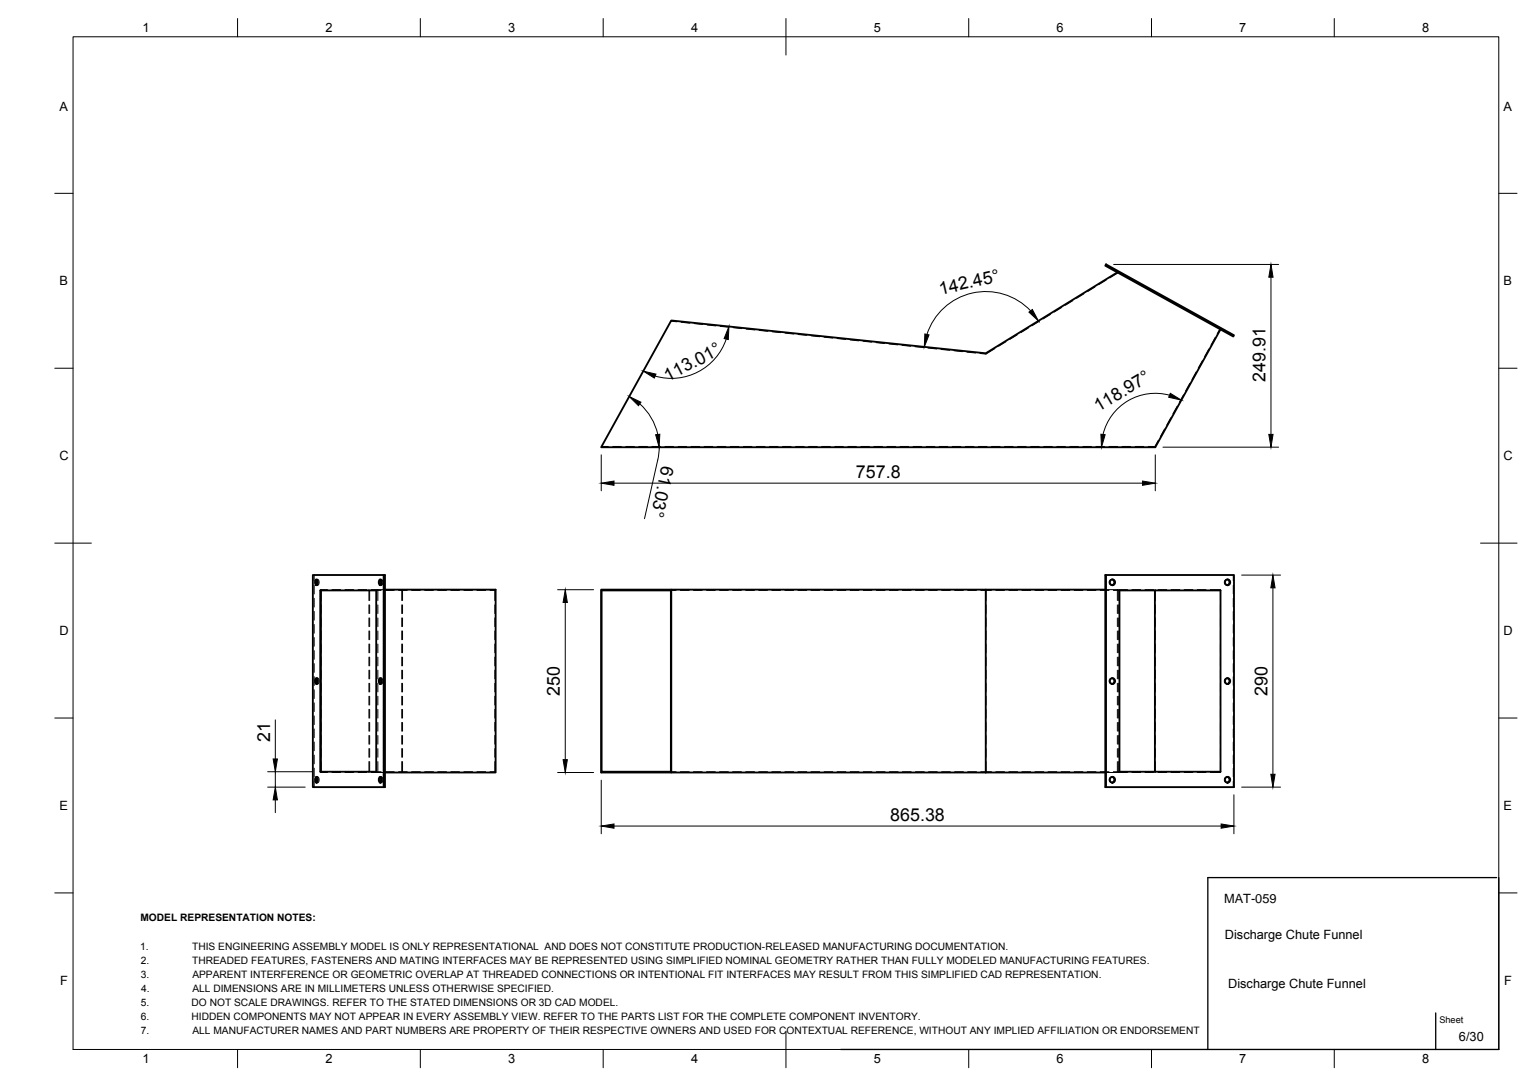
ISO-10303-21;
HEADER;
/* Generated by software containing ST-Developer
 * from STEP Tools, Inc. (www.steptools.com) 
 */

FILE_DESCRIPTION(
/* description */ ('', 'CAx-IF Rec.Pracs.---Representation and Presentation of Product Manufa
cturing Information (PMI)---4.0---2014-10-13'),
/* implementation_level */ '2;1');

FILE_NAME(
/* name */ 'Discharge Chute Funnel.step',
/* time_stamp */ '2026-10-28T23:00:48+01:00',
/* author */ (''),
/* organization */ (''),
/* preprocessor_version */ 'ST-DEVELOPER v20.2',
/* originating_system */ 'Autodesk Translation Framework v15.17.0.0',
/* authorisation */ '');

FILE_SCHEMA (('AP242_MANAGED_MODEL_BASED_3D_ENGINEERING_MIM_LF { 1 0 10303 442 2 1 4 }'));
ENDSEC;

DATA;
#10=MECHANICAL_DESIGN_GEOMETRIC_PRESENTATION_REPRESENTATION('',(#968),#61811);
#918=SHAPE_REPRESENTATION_RELATIONSHIP('SRR','None',#61976,#943);
#943=ADVANCED_BREP_SHAPE_REPRESENTATION('',(#1007),#61789);
#968=STYLED_ITEM('',(#62149),#1007);
#1007=MANIFOLD_SOLID_BREP('Body1',#33798);
#1101=CYLINDRICAL_SURFACE('',#34529,4.);
#1102=CYLINDRICAL_SURFACE('',#34532,4.);
#1103=CYLINDRICAL_SURFACE('',#34535,4.);
#1104=CYLINDRICAL_SURFACE('',#34538,4.);
#1105=CYLINDRICAL_SURFACE('',#34541,4.);
#1106=CYLINDRICAL_SURFACE('',#34544,4.);
#1908=FACE_BOUND('',#6367,.T.);
#1909=FACE_BOUND('',#6368,.T.);
#1910=FACE_BOUND('',#6369,.T.);
#1911=FACE_BOUND('',#6370,.T.);
#1912=FACE_BOUND('',#6371,.T.);
#1913=FACE_BOUND('',#6372,.T.);
#1914=FACE_BOUND('',#6373,.T.);
#1915=FACE_BOUND('',#6389,.T.);
#1916=FACE_BOUND('',#6390,.T.);
#1917=FACE_BOUND('',#6391,.T.);
#1918=FACE_BOUND('',#6392,.T.);
#1919=FACE_BOUND('',#6393,.T.);
#1920=FACE_BOUND('',#6394,.T.);
#1921=FACE_BOUND('',#6395,.T.);
#1922=FACE_BOUND('',#6399,.T.);
#2436=CIRCLE('',#34530,4.);
#2437=CIRCLE('',#34531,4.);
#2438=CIRCLE('',#34533,4.);
#2439=CIRCLE('',#34534,4.);
#2440=CIRCLE('',#34536,4.);
#2441=CIRCLE('',#34537,4.);
#2442=CIRCLE('',#34539,4.);
#2443=CIRCLE('',#34540,4.);
#2444=CIRCLE('',#34542,4.);
#2445=CIRCLE('',#34543,4.);
#2446=CIRCLE('',#34545,4.);
#2447=CIRCLE('',#34546,4.);
#4452=FACE_OUTER_BOUND('',#6360,.T.);
#4453=FACE_OUTER_BOUND('',#6361,.T.);
#4454=FACE_OUTER_BOUND('',#6362,.T.);
#4455=FACE_OUTER_BOUND('',#6363,.T.);
#4456=FACE_OUTER_BOUND('',#6364,.T.);
#4457=FACE_OUTER_BOUND('',#6365,.T.);
#4458=FACE_OUTER_BOUND('',#6366,.T.);
#4459=FACE_OUTER_BOUND('',#6374,.T.);
#4460=FACE_OUTER_BOUND('',#6375,.T.);
#4461=FACE_OUTER_BOUND('',#6376,.T.);
#4462=FACE_OUTER_BOUND('',#6377,.T.);
#4463=FACE_OUTER_BOUND('',#6378,.T.);
#4464=FACE_OUTER_BOUND('',#6379,.T.);
#4465=FACE_OUTER_BOUND('',#6380,.T.);
#4466=FACE_OUTER_BOUND('',#6381,.T.);
#4467=FACE_OUTER_BOUND('',#6382,.T.);
#4468=FACE_OUTER_BOUND('',#6383,.T.);
#4469=FACE_OUTER_BOUND('',#6384,.T.);
#4470=FACE_OUTER_BOUND('',#6385,.T.);
#4471=FACE_OUTER_BOUND('',#6386,.T.);
#4472=FACE_OUTER_BOUND('',#6387,.T.);
#4473=FACE_OUTER_BOUND('',#6388,.T.);
#4474=FACE_OUTER_BOUND('',#6396,.T.);
#4475=FACE_OUTER_BOUND('',#6397,.T.);
#4476=FACE_OUTER_BOUND('',#6398,.T.);
#4477=FACE_OUTER_BOUND('',#6400,.T.);
#4478=FACE_OUTER_BOUND('',#6401,.T.);
#6360=EDGE_LOOP('',(#22454,#22455,#22456,#22457));
#6361=EDGE_LOOP('',(#22458,#22459,#22460,#22461));
#6362=EDGE_LOOP('',(#22462,#22463,#22464,#22465));
#6363=EDGE_LOOP('',(#22466,#22467,#22468,#22469));
#6364=EDGE_LOOP('',(#22470,#22471,#22472,#22473));
#6365=EDGE_LOOP('',(#22474,#22475,#22476,#22477));
#6366=EDGE_LOOP('',(#22478,#22479,#22480,#22481));
#6367=EDGE_LOOP('',(#22482));
#6368=EDGE_LOOP('',(#22483));
#6369=EDGE_LOOP('',(#22484));
#6370=EDGE_LOOP('',(#22485));
#6371=EDGE_LOOP('',(#22486));
#6372=EDGE_LOOP('',(#22487));
#6373=EDGE_LOOP('',(#22488,#22489,#22490,#22491));
#6374=EDGE_LOOP('',(#22492,#22493,#22494,#22495));
#6375=EDGE_LOOP('',(#22496,#22497,#22498,#22499));
#6376=EDGE_LOOP('',(#22500,#22501,#22502,#22503));
#6377=EDGE_LOOP('',(#22504,#22505,#22506,#22507));
#6378=EDGE_LOOP('',(#22508,#22509,#22510,#22511));
#6379=EDGE_LOOP('',(#22512,#22513,#22514,#22515,#22516,#22517));
#6380=EDGE_LOOP('',(#22518,#22519,#22520,#22521));
#6381=EDGE_LOOP('',(#22522,#22523,#22524,#22525));
#6382=EDGE_LOOP('',(#22526,#22527,#22528,#22529));
#6383=EDGE_LOOP('',(#22530,#22531,#22532,#22533));
#6384=EDGE_LOOP('',(#22534,#22535,#22536,#22537));
#6385=EDGE_LOOP('',(#22538,#22539,#22540,#22541));
#6386=EDGE_LOOP('',(#22542,#22543,#22544,#22545,#22546,#22547,#22548,#22549));
#6387=EDGE_LOOP('',(#22550,#22551,#22552,#22553,#22554,#22555,#22556,#22557));
#6388=EDGE_LOOP('',(#22558,#22559,#22560,#22561));
#6389=EDGE_LOOP('',(#22562));
#6390=EDGE_LOOP('',(#22563));
#6391=EDGE_LOOP('',(#22564));
#6392=EDGE_LOOP('',(#22565));
#6393=EDGE_LOOP('',(#22566));
#6394=EDGE_LOOP('',(#22567));
#6395=EDGE_LOOP('',(#22568,#22569,#22570,#22571));
#6396=EDGE_LOOP('',(#22572,#22573,#22574,#22575));
#6397=EDGE_LOOP('',(#22576,#22577,#22578,#22579));
#6398=EDGE_LOOP('',(#22580,#22581,#22582,#22583));
#6399=EDGE_LOOP('',(#22584,#22585,#22586,#22587));
#6400=EDGE_LOOP('',(#22588,#22589,#22590,#22591));
#6401=EDGE_LOOP('',(#22592,#22593,#22594,#22595,#22596,#22597));
#8576=LINE('',#51421,#11123);
#8577=LINE('',#51427,#11124);
#8578=LINE('',#51433,#11125);
#8579=LINE('',#51439,#11126);
#8580=LINE('',#51445,#11127);
#8581=LINE('',#51451,#11128);
#8582=LINE('',#51456,#11129);
#8583=LINE('',#51458,#11130);
#8584=LINE('',#51460,#11131);
#8585=LINE('',#51461,#11132);
#8586=LINE('',#51464,#11133);
#8587=LINE('',#51466,#11134);
#8588=LINE('',#51468,#11135);
#8589=LINE('',#51469,#11136);
#8590=LINE('',#51473,#11137);
#8591=LINE('',#51474,#11138);
#8592=LINE('',#51475,#11139);
#8593=LINE('',#51478,#11140);
#8594=LINE('',#51479,#11141);
#8595=LINE('',#51482,#11142);
#8596=LINE('',#51483,#11143);
#8597=LINE('',#51485,#11144);
#8598=LINE('',#51488,#11145);
#8599=LINE('',#51490,#11146);
#8600=LINE('',#51491,#11147);
#8601=LINE('',#51494,#11148);
#8602=LINE('',#51496,#11149);
#8603=LINE('',#51498,#11150);
#8604=LINE('',#51499,#11151);
#8605=LINE('',#51503,#11152);
#8606=LINE('',#51505,#11153);
#8607=LINE('',#51507,#11154);
#8608=LINE('',#51508,#11155);
#8609=LINE('',#51511,#11156);
#8610=LINE('',#51513,#11157);
#8611=LINE('',#51514,#11158);
#8612=LINE('',#51518,#11159);
#8613=LINE('',#51520,#11160);
#8614=LINE('',#51522,#11161);
#8615=LINE('',#51523,#11162);
#8616=LINE('',#51526,#11163);
#8617=LINE('',#51528,#11164);
#8618=LINE('',#51529,#11165);
#8619=LINE('',#51532,#11166);
#8620=LINE('',#51534,#11167);
#8621=LINE('',#51535,#11168);
#8622=LINE('',#51538,#11169);
#8623=LINE('',#51540,#11170);
#8624=LINE('',#51541,#11171);
#8625=LINE('',#51543,#11172);
#8626=LINE('',#51544,#11173);
#8627=LINE('',#51546,#11174);
#8628=LINE('',#51547,#11175);
#8629=LINE('',#51551,#11176);
#8630=LINE('',#51552,#11177);
#8631=LINE('',#51555,#11178);
#8632=LINE('',#51556,#11179);
#8633=LINE('',#51559,#11180);
#8634=LINE('',#51560,#11181);
#8635=LINE('',#51562,#11182);
#11123=VECTOR('',#39234,4.);
#11124=VECTOR('',#39241,4.);
#11125=VECTOR('',#39248,4.);
#11126=VECTOR('',#39255,4.);
#11127=VECTOR('',#39262,4.);
#11128=VECTOR('',#39269,4.);
#11129=VECTOR('',#39274,10.);
#11130=VECTOR('',#39275,10.);
#11131=VECTOR('',#39276,10.);
#11132=VECTOR('',#39277,10.);
#11133=VECTOR('',#39278,10.);
#11134=VECTOR('',#39279,10.);
#11135=VECTOR('',#39280,10.);
#11136=VECTOR('',#39281,10.);
#11137=VECTOR('',#39284,10.);
#11138=VECTOR('',#39285,10.);
#11139=VECTOR('',#39286,10.);
#11140=VECTOR('',#39289,10.);
#11141=VECTOR('',#39290,10.);
#11142=VECTOR('',#39293,10.);
#11143=VECTOR('',#39294,10.);
#11144=VECTOR('',#39297,10.);
#11145=VECTOR('',#39300,10.);
#11146=VECTOR('',#39301,10.);
#11147=VECTOR('',#39302,10.);
#11148=VECTOR('',#39305,10.);
#11149=VECTOR('',#39306,10.);
#11150=VECTOR('',#39307,10.);
#11151=VECTOR('',#39308,10.);
#11152=VECTOR('',#39311,10.);
#11153=VECTOR('',#39312,10.);
#11154=VECTOR('',#39313,10.);
#11155=VECTOR('',#39314,10.);
#11156=VECTOR('',#39317,10.);
#11157=VECTOR('',#39318,10.);
#11158=VECTOR('',#39319,10.);
#11159=VECTOR('',#39322,10.);
#11160=VECTOR('',#39323,10.);
#11161=VECTOR('',#39324,10.);
#11162=VECTOR('',#39325,10.);
#11163=VECTOR('',#39328,10.);
#11164=VECTOR('',#39329,10.);
#11165=VECTOR('',#39330,10.);
#11166=VECTOR('',#39333,10.);
#11167=VECTOR('',#39334,10.);
#11168=VECTOR('',#39335,10.);
#11169=VECTOR('',#39338,10.);
#11170=VECTOR('',#39339,10.);
#11171=VECTOR('',#39340,10.);
#11172=VECTOR('',#39343,10.);
#11173=VECTOR('',#39344,10.);
#11174=VECTOR('',#39347,10.);
#11175=VECTOR('',#39348,10.);
#11176=VECTOR('',#39353,10.);
#11177=VECTOR('',#39354,10.);
#11178=VECTOR('',#39357,10.);
#11179=VECTOR('',#39358,10.);
#11180=VECTOR('',#39361,10.);
#11181=VECTOR('',#39362,10.);
#11182=VECTOR('',#39365,10.);
#13748=VERTEX_POINT('',#51418);
#13749=VERTEX_POINT('',#51420);
#13750=VERTEX_POINT('',#51424);
#13751=VERTEX_POINT('',#51426);
#13752=VERTEX_POINT('',#51430);
#13753=VERTEX_POINT('',#51432);
#13754=VERTEX_POINT('',#51436);
#13755=VERTEX_POINT('',#51438);
#13756=VERTEX_POINT('',#51442);
#13757=VERTEX_POINT('',#51444);
#13758=VERTEX_POINT('',#51448);
#13759=VERTEX_POINT('',#51450);
#13760=VERTEX_POINT('',#51454);
#13761=VERTEX_POINT('',#51455);
#13762=VERTEX_POINT('',#51457);
#13763=VERTEX_POINT('',#51459);
#13764=VERTEX_POINT('',#51462);
#13765=VERTEX_POINT('',#51463);
#13766=VERTEX_POINT('',#51465);
#13767=VERTEX_POINT('',#51467);
#13768=VERTEX_POINT('',#51471);
#13769=VERTEX_POINT('',#51472);
#13770=VERTEX_POINT('',#51477);
#13771=VERTEX_POINT('',#51481);
#13772=VERTEX_POINT('',#51487);
#13773=VERTEX_POINT('',#51489);
#13774=VERTEX_POINT('',#51493);
#13775=VERTEX_POINT('',#51495);
#13776=VERTEX_POINT('',#51497);
#13777=VERTEX_POINT('',#51501);
#13778=VERTEX_POINT('',#51502);
#13779=VERTEX_POINT('',#51504);
#13780=VERTEX_POINT('',#51506);
#13781=VERTEX_POINT('',#51510);
#13782=VERTEX_POINT('',#51512);
#13783=VERTEX_POINT('',#51516);
#13784=VERTEX_POINT('',#51517);
#13785=VERTEX_POINT('',#51519);
#13786=VERTEX_POINT('',#51521);
#13787=VERTEX_POINT('',#51525);
#13788=VERTEX_POINT('',#51527);
#13789=VERTEX_POINT('',#51531);
#13790=VERTEX_POINT('',#51533);
#13791=VERTEX_POINT('',#51537);
#13792=VERTEX_POINT('',#51539);
#13793=VERTEX_POINT('',#51550);
#13794=VERTEX_POINT('',#51554);
#13795=VERTEX_POINT('',#51558);
#17129=EDGE_CURVE('',#13748,#13748,#2436,.T.);
#17130=EDGE_CURVE('',#13748,#13749,#8576,.T.);
#17131=EDGE_CURVE('',#13749,#13749,#2437,.T.);
#17132=EDGE_CURVE('',#13750,#13750,#2438,.T.);
#17133=EDGE_CURVE('',#13750,#13751,#8577,.T.);
#17134=EDGE_CURVE('',#13751,#13751,#2439,.T.);
#17135=EDGE_CURVE('',#13752,#13752,#2440,.T.);
#17136=EDGE_CURVE('',#13752,#13753,#8578,.T.);
#17137=EDGE_CURVE('',#13753,#13753,#2441,.T.);
#17138=EDGE_CURVE('',#13754,#13754,#2442,.T.);
#17139=EDGE_CURVE('',#13754,#13755,#8579,.T.);
#17140=EDGE_CURVE('',#13755,#13755,#2443,.T.);
#17141=EDGE_CURVE('',#13756,#13756,#2444,.T.);
#17142=EDGE_CURVE('',#13756,#13757,#8580,.T.);
#17143=EDGE_CURVE('',#13757,#13757,#2445,.T.);
#17144=EDGE_CURVE('',#13758,#13758,#2446,.T.);
#17145=EDGE_CURVE('',#13758,#13759,#8581,.T.);
#17146=EDGE_CURVE('',#13759,#13759,#2447,.T.);
#17147=EDGE_CURVE('',#13760,#13761,#8582,.T.);
#17148=EDGE_CURVE('',#13761,#13762,#8583,.T.);
#17149=EDGE_CURVE('',#13762,#13763,#8584,.T.);
#17150=EDGE_CURVE('',#13763,#13760,#8585,.T.);
#17151=EDGE_CURVE('',#13764,#13765,#8586,.T.);
#17152=EDGE_CURVE('',#13766,#13764,#8587,.T.);
#17153=EDGE_CURVE('',#13767,#13766,#8588,.T.);
#17154=EDGE_CURVE('',#13765,#13767,#8589,.T.);
#17155=EDGE_CURVE('',#13768,#13769,#8590,.T.);
#17156=EDGE_CURVE('',#13769,#13760,#8591,.T.);
#17157=EDGE_CURVE('',#13768,#13763,#8592,.T.);
#17158=EDGE_CURVE('',#13770,#13768,#8593,.T.);
#17159=EDGE_CURVE('',#13770,#13762,#8594,.T.);
#17160=EDGE_CURVE('',#13771,#13770,#8595,.T.);
#17161=EDGE_CURVE('',#13771,#13761,#8596,.T.);
#17162=EDGE_CURVE('',#13769,#13771,#8597,.T.);
#17163=EDGE_CURVE('',#13767,#13772,#8598,.T.);
#17164=EDGE_CURVE('',#13772,#13773,#8599,.T.);
#17165=EDGE_CURVE('',#13765,#13773,#8600,.T.);
#17166=EDGE_CURVE('',#13774,#13766,#8601,.T.);
#17167=EDGE_CURVE('',#13775,#13774,#8602,.T.);
#17168=EDGE_CURVE('',#13776,#13775,#8603,.T.);
#17169=EDGE_CURVE('',#13772,#13776,#8604,.T.);
#17170=EDGE_CURVE('',#13777,#13778,#8605,.T.);
#17171=EDGE_CURVE('',#13779,#13777,#8606,.T.);
#17172=EDGE_CURVE('',#13780,#13779,#8607,.T.);
#17173=EDGE_CURVE('',#13780,#13778,#8608,.T.);
#17174=EDGE_CURVE('',#13781,#13778,#8609,.T.);
#17175=EDGE_CURVE('',#13781,#13782,#8610,.F.);
#17176=EDGE_CURVE('',#13782,#13777,#8611,.T.);
#17177=EDGE_CURVE('',#13783,#13784,#8612,.T.);
#17178=EDGE_CURVE('',#13785,#13784,#8613,.T.);
#17179=EDGE_CURVE('',#13786,#13785,#8614,.T.);
#17180=EDGE_CURVE('',#13783,#13786,#8615,.T.);
#17181=EDGE_CURVE('',#13787,#13782,#8616,.T.);
#17182=EDGE_CURVE('',#13788,#13781,#8617,.T.);
#17183=EDGE_CURVE('',#13788,#13787,#8618,.T.);
#17184=EDGE_CURVE('',#13789,#13787,#8619,.T.);
#17185=EDGE_CURVE('',#13790,#13788,#8620,.T.);
#17186=EDGE_CURVE('',#13789,#13790,#8621,.T.);
#17187=EDGE_CURVE('',#13784,#13791,#8622,.T.);
#17188=EDGE_CURVE('',#13792,#13791,#8623,.T.);
#17189=EDGE_CURVE('',#13785,#13792,#8624,.T.);
#17190=EDGE_CURVE('',#13790,#13792,#8625,.T.);
#17191=EDGE_CURVE('',#13786,#13780,#8626,.T.);
#17192=EDGE_CURVE('',#13791,#13789,#8627,.T.);
#17193=EDGE_CURVE('',#13779,#13783,#8628,.T.);
#17194=EDGE_CURVE('',#13793,#13764,#8629,.T.);
#17195=EDGE_CURVE('',#13774,#13793,#8630,.T.);
#17196=EDGE_CURVE('',#13794,#13793,#8631,.T.);
#17197=EDGE_CURVE('',#13775,#13794,#8632,.T.);
#17198=EDGE_CURVE('',#13795,#13794,#8633,.T.);
#17199=EDGE_CURVE('',#13776,#13795,#8634,.T.);
#17200=EDGE_CURVE('',#13773,#13795,#8635,.T.);
#22454=ORIENTED_EDGE('',*,*,#17129,.F.);
#22455=ORIENTED_EDGE('',*,*,#17130,.T.);
#22456=ORIENTED_EDGE('',*,*,#17131,.F.);
#22457=ORIENTED_EDGE('',*,*,#17130,.F.);
#22458=ORIENTED_EDGE('',*,*,#17132,.F.);
#22459=ORIENTED_EDGE('',*,*,#17133,.T.);
#22460=ORIENTED_EDGE('',*,*,#17134,.F.);
#22461=ORIENTED_EDGE('',*,*,#17133,.F.);
#22462=ORIENTED_EDGE('',*,*,#17135,.F.);
#22463=ORIENTED_EDGE('',*,*,#17136,.T.);
#22464=ORIENTED_EDGE('',*,*,#17137,.F.);
#22465=ORIENTED_EDGE('',*,*,#17136,.F.);
#22466=ORIENTED_EDGE('',*,*,#17138,.F.);
#22467=ORIENTED_EDGE('',*,*,#17139,.T.);
#22468=ORIENTED_EDGE('',*,*,#17140,.F.);
#22469=ORIENTED_EDGE('',*,*,#17139,.F.);
#22470=ORIENTED_EDGE('',*,*,#17141,.F.);
#22471=ORIENTED_EDGE('',*,*,#17142,.T.);
#22472=ORIENTED_EDGE('',*,*,#17143,.F.);
#22473=ORIENTED_EDGE('',*,*,#17142,.F.);
#22474=ORIENTED_EDGE('',*,*,#17144,.F.);
#22475=ORIENTED_EDGE('',*,*,#17145,.T.);
#22476=ORIENTED_EDGE('',*,*,#17146,.F.);
#22477=ORIENTED_EDGE('',*,*,#17145,.F.);
#22478=ORIENTED_EDGE('',*,*,#17147,.T.);
#22479=ORIENTED_EDGE('',*,*,#17148,.T.);
#22480=ORIENTED_EDGE('',*,*,#17149,.T.);
#22481=ORIENTED_EDGE('',*,*,#17150,.T.);
#22482=ORIENTED_EDGE('',*,*,#17131,.T.);
#22483=ORIENTED_EDGE('',*,*,#17134,.T.);
#22484=ORIENTED_EDGE('',*,*,#17137,.T.);
#22485=ORIENTED_EDGE('',*,*,#17140,.T.);
#22486=ORIENTED_EDGE('',*,*,#17143,.T.);
#22487=ORIENTED_EDGE('',*,*,#17146,.T.);
#22488=ORIENTED_EDGE('',*,*,#17151,.F.);
#22489=ORIENTED_EDGE('',*,*,#17152,.F.);
#22490=ORIENTED_EDGE('',*,*,#17153,.F.);
#22491=ORIENTED_EDGE('',*,*,#17154,.F.);
#22492=ORIENTED_EDGE('',*,*,#17155,.T.);
#22493=ORIENTED_EDGE('',*,*,#17156,.T.);
#22494=ORIENTED_EDGE('',*,*,#17150,.F.);
#22495=ORIENTED_EDGE('',*,*,#17157,.F.);
#22496=ORIENTED_EDGE('',*,*,#17158,.T.);
#22497=ORIENTED_EDGE('',*,*,#17157,.T.);
#22498=ORIENTED_EDGE('',*,*,#17149,.F.);
#22499=ORIENTED_EDGE('',*,*,#17159,.F.);
#22500=ORIENTED_EDGE('',*,*,#17160,.T.);
#22501=ORIENTED_EDGE('',*,*,#17159,.T.);
#22502=ORIENTED_EDGE('',*,*,#17148,.F.);
#22503=ORIENTED_EDGE('',*,*,#17161,.F.);
#22504=ORIENTED_EDGE('',*,*,#17162,.T.);
#22505=ORIENTED_EDGE('',*,*,#17161,.T.);
#22506=ORIENTED_EDGE('',*,*,#17147,.F.);
#22507=ORIENTED_EDGE('',*,*,#17156,.F.);
#22508=ORIENTED_EDGE('',*,*,#17154,.T.);
#22509=ORIENTED_EDGE('',*,*,#17163,.T.);
#22510=ORIENTED_EDGE('',*,*,#17164,.T.);
#22511=ORIENTED_EDGE('',*,*,#17165,.F.);
#22512=ORIENTED_EDGE('',*,*,#17153,.T.);
#22513=ORIENTED_EDGE('',*,*,#17166,.F.);
#22514=ORIENTED_EDGE('',*,*,#17167,.F.);
#22515=ORIENTED_EDGE('',*,*,#17168,.F.);
#22516=ORIENTED_EDGE('',*,*,#17169,.F.);
#22517=ORIENTED_EDGE('',*,*,#17163,.F.);
#22518=ORIENTED_EDGE('',*,*,#17170,.F.);
#22519=ORIENTED_EDGE('',*,*,#17171,.F.);
#22520=ORIENTED_EDGE('',*,*,#17172,.F.);
#22521=ORIENTED_EDGE('',*,*,#17173,.T.);
#22522=ORIENTED_EDGE('',*,*,#17170,.T.);
#22523=ORIENTED_EDGE('',*,*,#17174,.F.);
#22524=ORIENTED_EDGE('',*,*,#17175,.T.);
#22525=ORIENTED_EDGE('',*,*,#17176,.T.);
#22526=ORIENTED_EDGE('',*,*,#17177,.T.);
#22527=ORIENTED_EDGE('',*,*,#17178,.F.);
#22528=ORIENTED_EDGE('',*,*,#17179,.F.);
#22529=ORIENTED_EDGE('',*,*,#17180,.F.);
#22530=ORIENTED_EDGE('',*,*,#17181,.T.);
#22531=ORIENTED_EDGE('',*,*,#17175,.F.);
#22532=ORIENTED_EDGE('',*,*,#17182,.F.);
#22533=ORIENTED_EDGE('',*,*,#17183,.T.);
#22534=ORIENTED_EDGE('',*,*,#17184,.T.);
#22535=ORIENTED_EDGE('',*,*,#17183,.F.);
#22536=ORIENTED_EDGE('',*,*,#17185,.F.);
#22537=ORIENTED_EDGE('',*,*,#17186,.F.);
#22538=ORIENTED_EDGE('',*,*,#17187,.T.);
#22539=ORIENTED_EDGE('',*,*,#17188,.F.);
#22540=ORIENTED_EDGE('',*,*,#17189,.F.);
#22541=ORIENTED_EDGE('',*,*,#17178,.T.);
#22542=ORIENTED_EDGE('',*,*,#17179,.T.);
#22543=ORIENTED_EDGE('',*,*,#17189,.T.);
#22544=ORIENTED_EDGE('',*,*,#17190,.F.);
#22545=ORIENTED_EDGE('',*,*,#17185,.T.);
#22546=ORIENTED_EDGE('',*,*,#17182,.T.);
#22547=ORIENTED_EDGE('',*,*,#17174,.T.);
#22548=ORIENTED_EDGE('',*,*,#17173,.F.);
#22549=ORIENTED_EDGE('',*,*,#17191,.F.);
#22550=ORIENTED_EDGE('',*,*,#17176,.F.);
#22551=ORIENTED_EDGE('',*,*,#17181,.F.);
#22552=ORIENTED_EDGE('',*,*,#17184,.F.);
#22553=ORIENTED_EDGE('',*,*,#17192,.F.);
#22554=ORIENTED_EDGE('',*,*,#17187,.F.);
#22555=ORIENTED_EDGE('',*,*,#17177,.F.);
#22556=ORIENTED_EDGE('',*,*,#17193,.F.);
#22557=ORIENTED_EDGE('',*,*,#17171,.T.);
#22558=ORIENTED_EDGE('',*,*,#17162,.F.);
#22559=ORIENTED_EDGE('',*,*,#17155,.F.);
#22560=ORIENTED_EDGE('',*,*,#17158,.F.);
#22561=ORIENTED_EDGE('',*,*,#17160,.F.);
#22562=ORIENTED_EDGE('',*,*,#17129,.T.);
#22563=ORIENTED_EDGE('',*,*,#17132,.T.);
#22564=ORIENTED_EDGE('',*,*,#17135,.T.);
#22565=ORIENTED_EDGE('',*,*,#17138,.T.);
#22566=ORIENTED_EDGE('',*,*,#17141,.T.);
#22567=ORIENTED_EDGE('',*,*,#17144,.T.);
#22568=ORIENTED_EDGE('',*,*,#17180,.T.);
#22569=ORIENTED_EDGE('',*,*,#17191,.T.);
#22570=ORIENTED_EDGE('',*,*,#17172,.T.);
#22571=ORIENTED_EDGE('',*,*,#17193,.T.);
#22572=ORIENTED_EDGE('',*,*,#17152,.T.);
#22573=ORIENTED_EDGE('',*,*,#17194,.F.);
#22574=ORIENTED_EDGE('',*,*,#17195,.F.);
#22575=ORIENTED_EDGE('',*,*,#17166,.T.);
#22576=ORIENTED_EDGE('',*,*,#17196,.F.);
#22577=ORIENTED_EDGE('',*,*,#17197,.F.);
#22578=ORIENTED_EDGE('',*,*,#17167,.T.);
#22579=ORIENTED_EDGE('',*,*,#17195,.T.);
#22580=ORIENTED_EDGE('',*,*,#17198,.F.);
#22581=ORIENTED_EDGE('',*,*,#17199,.F.);
#22582=ORIENTED_EDGE('',*,*,#17168,.T.);
#22583=ORIENTED_EDGE('',*,*,#17197,.T.);
#22584=ORIENTED_EDGE('',*,*,#17188,.T.);
#22585=ORIENTED_EDGE('',*,*,#17192,.T.);
#22586=ORIENTED_EDGE('',*,*,#17186,.T.);
#22587=ORIENTED_EDGE('',*,*,#17190,.T.);
#22588=ORIENTED_EDGE('',*,*,#17200,.F.);
#22589=ORIENTED_EDGE('',*,*,#17164,.F.);
#22590=ORIENTED_EDGE('',*,*,#17169,.T.);
#22591=ORIENTED_EDGE('',*,*,#17199,.T.);
#22592=ORIENTED_EDGE('',*,*,#17151,.T.);
#22593=ORIENTED_EDGE('',*,*,#17165,.T.);
#22594=ORIENTED_EDGE('',*,*,#17200,.T.);
#22595=ORIENTED_EDGE('',*,*,#17198,.T.);
#22596=ORIENTED_EDGE('',*,*,#17196,.T.);
#22597=ORIENTED_EDGE('',*,*,#17194,.T.);
#31203=PLANE('',#34547);
#31204=PLANE('',#34548);
#31205=PLANE('',#34549);
#31206=PLANE('',#34550);
#31207=PLANE('',#34551);
#31208=PLANE('',#34552);
#31209=PLANE('',#34553);
#31210=PLANE('',#34554);
#31211=PLANE('',#34555);
#31212=PLANE('',#34556);
#31213=PLANE('',#34557);
#31214=PLANE('',#34558);
#31215=PLANE('',#34559);
#31216=PLANE('',#34560);
#31217=PLANE('',#34561);
#31218=PLANE('',#34562);
#31219=PLANE('',#34563);
#31220=PLANE('',#34564);
#31221=PLANE('',#34565);
#31222=PLANE('',#34566);
#31223=PLANE('',#34567);
#32133=ADVANCED_FACE('',(#4452),#1101,.F.);
#32134=ADVANCED_FACE('',(#4453),#1102,.F.);
#32135=ADVANCED_FACE('',(#4454),#1103,.F.);
#32136=ADVANCED_FACE('',(#4455),#1104,.F.);
#32137=ADVANCED_FACE('',(#4456),#1105,.F.);
#32138=ADVANCED_FACE('',(#4457),#1106,.F.);
#32139=ADVANCED_FACE('',(#4458,#1908,#1909,#1910,#1911,#1912,#1913,#1914),
#31203,.T.);
#32140=ADVANCED_FACE('',(#4459),#31204,.T.);
#32141=ADVANCED_FACE('',(#4460),#31205,.T.);
#32142=ADVANCED_FACE('',(#4461),#31206,.T.);
#32143=ADVANCED_FACE('',(#4462),#31207,.T.);
#32144=ADVANCED_FACE('',(#4463),#31208,.T.);
#32145=ADVANCED_FACE('',(#4464),#31209,.T.);
#32146=ADVANCED_FACE('',(#4465),#31210,.F.);
#32147=ADVANCED_FACE('',(#4466),#31211,.F.);
#32148=ADVANCED_FACE('',(#4467),#31212,.F.);
#32149=ADVANCED_FACE('',(#4468),#31213,.F.);
#32150=ADVANCED_FACE('',(#4469),#31214,.F.);
#32151=ADVANCED_FACE('',(#4470),#31215,.F.);
#32152=ADVANCED_FACE('',(#4471),#31216,.F.);
#32153=ADVANCED_FACE('',(#4472),#31217,.T.);
#32154=ADVANCED_FACE('',(#4473,#1915,#1916,#1917,#1918,#1919,#1920,#1921),
#31218,.T.);
#32155=ADVANCED_FACE('',(#4474),#31219,.T.);
#32156=ADVANCED_FACE('',(#4475),#31220,.T.);
#32157=ADVANCED_FACE('',(#4476,#1922),#31221,.T.);
#32158=ADVANCED_FACE('',(#4477),#31222,.T.);
#32159=ADVANCED_FACE('',(#4478),#31223,.F.);
#33798=CLOSED_SHELL('',(#32133,#32134,#32135,#32136,#32137,#32138,#32139,
#32140,#32141,#32142,#32143,#32144,#32145,#32146,#32147,#32148,#32149,#32150,
#32151,#32152,#32153,#32154,#32155,#32156,#32157,#32158,#32159));
#34528=AXIS2_PLACEMENT_3D('',#51416,#39228,#39229);
#34529=AXIS2_PLACEMENT_3D('',#51417,#39230,#39231);
#34530=AXIS2_PLACEMENT_3D('',#51419,#39232,#39233);
#34531=AXIS2_PLACEMENT_3D('',#51422,#39235,#39236);
#34532=AXIS2_PLACEMENT_3D('',#51423,#39237,#39238);
#34533=AXIS2_PLACEMENT_3D('',#51425,#39239,#39240);
#34534=AXIS2_PLACEMENT_3D('',#51428,#39242,#39243);
#34535=AXIS2_PLACEMENT_3D('',#51429,#39244,#39245);
#34536=AXIS2_PLACEMENT_3D('',#51431,#39246,#39247);
#34537=AXIS2_PLACEMENT_3D('',#51434,#39249,#39250);
#34538=AXIS2_PLACEMENT_3D('',#51435,#39251,#39252);
#34539=AXIS2_PLACEMENT_3D('',#51437,#39253,#39254);
#34540=AXIS2_PLACEMENT_3D('',#51440,#39256,#39257);
#34541=AXIS2_PLACEMENT_3D('',#51441,#39258,#39259);
#34542=AXIS2_PLACEMENT_3D('',#51443,#39260,#39261);
#34543=AXIS2_PLACEMENT_3D('',#51446,#39263,#39264);
#34544=AXIS2_PLACEMENT_3D('',#51447,#39265,#39266);
#34545=AXIS2_PLACEMENT_3D('',#51449,#39267,#39268);
#34546=AXIS2_PLACEMENT_3D('',#51452,#39270,#39271);
#34547=AXIS2_PLACEMENT_3D('',#51453,#39272,#39273);
#34548=AXIS2_PLACEMENT_3D('',#51470,#39282,#39283);
#34549=AXIS2_PLACEMENT_3D('',#51476,#39287,#39288);
#34550=AXIS2_PLACEMENT_3D('',#51480,#39291,#39292);
#34551=AXIS2_PLACEMENT_3D('',#51484,#39295,#39296);
#34552=AXIS2_PLACEMENT_3D('',#51486,#39298,#39299);
#34553=AXIS2_PLACEMENT_3D('',#51492,#39303,#39304);
#34554=AXIS2_PLACEMENT_3D('',#51500,#39309,#39310);
#34555=AXIS2_PLACEMENT_3D('',#51509,#39315,#39316);
#34556=AXIS2_PLACEMENT_3D('',#51515,#39320,#39321);
#34557=AXIS2_PLACEMENT_3D('',#51524,#39326,#39327);
#34558=AXIS2_PLACEMENT_3D('',#51530,#39331,#39332);
#34559=AXIS2_PLACEMENT_3D('',#51536,#39336,#39337);
#34560=AXIS2_PLACEMENT_3D('',#51542,#39341,#39342);
#34561=AXIS2_PLACEMENT_3D('',#51545,#39345,#39346);
#34562=AXIS2_PLACEMENT_3D('',#51548,#39349,#39350);
#34563=AXIS2_PLACEMENT_3D('',#51549,#39351,#39352);
#34564=AXIS2_PLACEMENT_3D('',#51553,#39355,#39356);
#34565=AXIS2_PLACEMENT_3D('',#51557,#39359,#39360);
#34566=AXIS2_PLACEMENT_3D('',#51561,#39363,#39364);
#34567=AXIS2_PLACEMENT_3D('',#51563,#39366,#39367);
#39228=DIRECTION('axis',(0.,0.,1.));
#39229=DIRECTION('refdir',(1.,0.,0.));
#39230=DIRECTION('center_axis',(-3.34404360992166E-15,6.19091607821767E-16,
-1.));
#39231=DIRECTION('ref_axis',(-5.00596043936355E-16,-1.,-6.19091607821765E-16));
#39232=DIRECTION('center_axis',(-3.34404360992166E-15,6.19091607821767E-16,
-1.));
#39233=DIRECTION('ref_axis',(-5.00596043936355E-16,-1.,-6.19091607821765E-16));
#39234=DIRECTION('',(-3.34404360992166E-15,6.19091607821767E-16,-1.));
#39235=DIRECTION('center_axis',(3.34404360992166E-15,-6.19091607821767E-16,
1.));
#39236=DIRECTION('ref_axis',(-5.00596043936355E-16,-1.,-6.19091607821765E-16));
#39237=DIRECTION('center_axis',(-3.34404360992166E-15,6.19091607821767E-16,
-1.));
#39238=DIRECTION('ref_axis',(-5.00596043936355E-16,-1.,-6.19091607821765E-16));
#39239=DIRECTION('center_axis',(-3.34404360992166E-15,6.19091607821767E-16,
-1.));
#39240=DIRECTION('ref_axis',(-5.00596043936355E-16,-1.,-6.19091607821765E-16));
#39241=DIRECTION('',(-3.34404360992166E-15,6.19091607821767E-16,-1.));
#39242=DIRECTION('center_axis',(3.34404360992166E-15,-6.19091607821767E-16,
1.));
#39243=DIRECTION('ref_axis',(-5.00596043936355E-16,-1.,-6.19091607821765E-16));
#39244=DIRECTION('center_axis',(-3.34404360992166E-15,6.19091607821767E-16,
-1.));
#39245=DIRECTION('ref_axis',(-5.00596043936355E-16,-1.,-6.19091607821765E-16));
#39246=DIRECTION('center_axis',(-3.34404360992166E-15,6.19091607821767E-16,
-1.));
#39247=DIRECTION('ref_axis',(-5.00596043936355E-16,-1.,-6.19091607821765E-16));
#39248=DIRECTION('',(-3.34404360992166E-15,6.19091607821767E-16,-1.));
#39249=DIRECTION('center_axis',(3.34404360992166E-15,-6.19091607821767E-16,
1.));
#39250=DIRECTION('ref_axis',(-5.00596043936355E-16,-1.,-6.19091607821765E-16));
#39251=DIRECTION('center_axis',(-3.34404360992166E-15,6.19091607821767E-16,
-1.));
#39252=DIRECTION('ref_axis',(-5.00596043936355E-16,-1.,-6.19091607821765E-16));
#39253=DIRECTION('center_axis',(-3.34404360992166E-15,6.19091607821767E-16,
-1.));
#39254=DIRECTION('ref_axis',(-5.00596043936355E-16,-1.,-6.19091607821765E-16));
#39255=DIRECTION('',(-3.34404360992166E-15,6.19091607821767E-16,-1.));
#39256=DIRECTION('center_axis',(3.34404360992166E-15,-6.19091607821767E-16,
1.));
#39257=DIRECTION('ref_axis',(-5.00596043936355E-16,-1.,-6.19091607821765E-16));
#39258=DIRECTION('center_axis',(-3.34404360992166E-15,6.19091607821767E-16,
-1.));
#39259=DIRECTION('ref_axis',(-5.00596043936355E-16,-1.,-6.19091607821765E-16));
#39260=DIRECTION('center_axis',(-3.34404360992166E-15,6.19091607821767E-16,
-1.));
#39261=DIRECTION('ref_axis',(-5.00596043936355E-16,-1.,-6.19091607821765E-16));
#39262=DIRECTION('',(-3.34404360992166E-15,6.19091607821767E-16,-1.));
#39263=DIRECTION('center_axis',(3.34404360992166E-15,-6.19091607821767E-16,
1.));
#39264=DIRECTION('ref_axis',(-5.00596043936355E-16,-1.,-6.19091607821765E-16));
#39265=DIRECTION('center_axis',(-3.34404360992166E-15,6.19091607821767E-16,
-1.));
#39266=DIRECTION('ref_axis',(-5.00596043936355E-16,-1.,-6.19091607821765E-16));
#39267=DIRECTION('center_axis',(-3.34404360992166E-15,6.19091607821767E-16,
-1.));
#39268=DIRECTION('ref_axis',(-5.00596043936355E-16,-1.,-6.19091607821765E-16));
#39269=DIRECTION('',(-3.34404360992166E-15,6.19091607821767E-16,-1.));
#39270=DIRECTION('center_axis',(3.34404360992166E-15,-6.19091607821767E-16,
1.));
#39271=DIRECTION('ref_axis',(-5.00596043936355E-16,-1.,-6.19091607821765E-16));
#39272=DIRECTION('center_axis',(-3.34404360992166E-15,6.19091607821767E-16,
-1.));
#39273=DIRECTION('ref_axis',(-5.00596043936355E-16,-1.,-6.19091607821765E-16));
#39274=DIRECTION('',(5.00596043936355E-16,1.,6.19091607821765E-16));
#39275=DIRECTION('',(1.,-5.00596043936353E-16,-3.34404360992166E-15));
#39276=DIRECTION('',(-5.00596043936355E-16,-1.,-6.19091607821765E-16));
#39277=DIRECTION('',(-1.,5.00596043936353E-16,3.34404360992166E-15));
#39278=DIRECTION('',(-5.00596043934461E-16,-1.,-6.19091607821765E-16));
#39279=DIRECTION('',(1.,-5.00596043936353E-16,-3.34404360992166E-15));
#39280=DIRECTION('',(5.00596043936355E-16,1.,6.19091607821765E-16));
#39281=DIRECTION('',(-1.,5.00596043936353E-16,3.34404360992166E-15));
#39282=DIRECTION('center_axis',(-5.00596043936355E-16,-1.,-6.19091607821765E-16));
#39283=DIRECTION('ref_axis',(-1.,5.00596043936353E-16,3.34404360992166E-15));
#39284=DIRECTION('',(-1.,5.00596043936353E-16,3.34404360992166E-15));
#39285=DIRECTION('',(-3.34404360992166E-15,6.19091607821767E-16,-1.));
#39286=DIRECTION('',(-3.34404360992166E-15,6.19091607821767E-16,-1.));
#39287=DIRECTION('center_axis',(1.,-5.00596043936353E-16,-3.34404360992166E-15));
#39288=DIRECTION('ref_axis',(-5.00596043936355E-16,-1.,-6.19091607821765E-16));
#39289=DIRECTION('',(-5.00596043936355E-16,-1.,-6.19091607821765E-16));
#39290=DIRECTION('',(-3.34404360992166E-15,6.19091607821767E-16,-1.));
#39291=DIRECTION('center_axis',(5.00596043936355E-16,1.,6.19091607821765E-16));
#39292=DIRECTION('ref_axis',(1.,-5.00596043936353E-16,-3.34404360992166E-15));
#39293=DIRECTION('',(1.,-5.00596043936353E-16,-3.34404360992166E-15));
#39294=DIRECTION('',(-3.34404360992166E-15,6.19091607821767E-16,-1.));
#39295=DIRECTION('center_axis',(-1.,5.00596043936353E-16,3.34404360992166E-15));
#39296=DIRECTION('ref_axis',(5.00596043936355E-16,1.,6.19091607821765E-16));
#39297=DIRECTION('',(5.00596043936355E-16,1.,6.19091607821765E-16));
#39298=DIRECTION('center_axis',(-5.00596043934278E-16,-1.,6.20455933714055E-13));
#39299=DIRECTION('ref_axis',(-3.34404360992197E-15,-6.20455933714055E-13,
-1.));
#39300=DIRECTION('',(-3.34404360992197E-15,-6.20455933714055E-13,-1.));
#39301=DIRECTION('',(1.,-5.00596043936353E-16,-3.34404360992166E-15));
#39302=DIRECTION('',(-3.34404360992226E-15,-6.20455933714055E-13,-1.));
#39303=DIRECTION('center_axis',(-1.,5.00596043936353E-16,3.34404360992166E-15));
#39304=DIRECTION('ref_axis',(-5.00596043936355E-16,-1.,-6.19091607821765E-16));
#39305=DIRECTION('',(2.66598427033833E-15,-0.491594368037543,0.870824309096714));
#39306=DIRECTION('',(8.46232198011949E-16,-0.920455750162943,0.390846788386413));
#39307=DIRECTION('',(3.34404360992196E-15,5.89417440552492E-13,1.));
#39308=DIRECTION('',(-1.18154003924372E-15,0.874903192709269,-0.484297845738681));
#39309=DIRECTION('center_axis',(5.00596043936355E-16,1.,6.19091607821765E-16));
#39310=DIRECTION('ref_axis',(1.,-5.00596043936353E-16,-3.34404360992166E-15));
#39311=DIRECTION('',(-1.,5.00596043936353E-16,3.34404360992166E-15));
#39312=DIRECTION('',(-3.34404360992166E-15,6.19091607821767E-16,-1.));
#39313=DIRECTION('',(1.,-5.00596043936353E-16,-3.34404360992166E-15));
#39314=DIRECTION('',(-3.34404360992166E-15,6.19091607821767E-16,-1.));
#39315=DIRECTION('center_axis',(3.34404360992166E-15,-6.19091607821767E-16,
1.));
#39316=DIRECTION('ref_axis',(-5.00596043936355E-16,-1.,-6.19091607821765E-16));
#39317=DIRECTION('',(-5.00596043936355E-16,-1.,-6.19091607821765E-16));
#39318=DIRECTION('',(-1.,5.00596043936353E-16,3.34404360992166E-15));
#39319=DIRECTION('',(-5.00596043934461E-16,-1.,-6.19091607821765E-16));
#39320=DIRECTION('center_axis',(-5.00596043934278E-16,-1.,6.20455933714055E-13));
#39321=DIRECTION('ref_axis',(-3.34404360992197E-15,-6.20455933714055E-13,
-1.));
#39322=DIRECTION('',(-3.34404360992226E-15,-6.20455933714055E-13,-1.));
#39323=DIRECTION('',(1.,-5.00596043936353E-16,-3.34404360992166E-15));
#39324=DIRECTION('',(-3.34404360992197E-15,-6.20455933714055E-13,-1.));
#39325=DIRECTION('',(-1.,5.00596043936353E-16,3.34404360992166E-15));
#39326=DIRECTION('center_axis',(2.07984420920684E-15,0.870824309096714,
0.491594368037543));
#39327=DIRECTION('ref_axis',(2.66598427033833E-15,-0.491594368037543,0.870824309096714));
#39328=DIRECTION('',(2.66598427033951E-15,-0.491594368037543,0.870824309096714));
#39329=DIRECTION('',(2.66598427033833E-15,-0.491594368037543,0.870824309096714));
#39330=DIRECTION('',(1.,-5.00596043936353E-16,-3.34404360992166E-15));
#39331=DIRECTION('center_axis',(3.27370052559951E-15,0.390846788386413,
0.920455750162943));
#39332=DIRECTION('ref_axis',(8.46232198011949E-16,-0.920455750162943,0.390846788386413));
#39333=DIRECTION('',(8.46232198013806E-16,-0.920455750162943,0.390846788386413));
#39334=DIRECTION('',(8.46232198011949E-16,-0.920455750162943,0.390846788386413));
#39335=DIRECTION('',(-1.,5.00596043936353E-16,3.34404360992166E-15));
#39336=DIRECTION('center_axis',(-3.16815201654317E-15,-0.484297845738681,
-0.874903192709269));
#39337=DIRECTION('ref_axis',(-1.18154003924372E-15,0.874903192709269,-0.484297845738681));
#39338=DIRECTION('',(-1.18154003924552E-15,0.874903192709269,-0.484297845738681));
#39339=DIRECTION('',(1.,-5.00596043936353E-16,-3.34404360992166E-15));
#39340=DIRECTION('',(-1.18154003924372E-15,0.874903192709269,-0.484297845738681));
#39341=DIRECTION('center_axis',(-1.,5.00596043936353E-16,3.34404360992166E-15));
#39342=DIRECTION('ref_axis',(-5.00596043936355E-16,-1.,-6.19091607821765E-16));
#39343=DIRECTION('',(-3.34404360992196E-15,-5.89417440552492E-13,-1.));
#39344=DIRECTION('',(5.00596043936355E-16,1.,6.19091607821765E-16));
#39345=DIRECTION('center_axis',(-1.,5.00596043934459E-16,3.34404360992195E-15));
#39346=DIRECTION('ref_axis',(-5.00596043934461E-16,-1.,-6.19091607821765E-16));
#39347=DIRECTION('',(3.34404360992225E-15,5.89417440552492E-13,1.));
#39348=DIRECTION('',(-5.00596043936355E-16,-1.,-6.19091607821765E-16));
#39349=DIRECTION('center_axis',(3.34404360992166E-15,-6.19091607821767E-16,
1.));
#39350=DIRECTION('ref_axis',(-5.00596043936355E-16,-1.,-6.19091607821765E-16));
#39351=DIRECTION('center_axis',(2.07984420920684E-15,0.870824309096714,
0.491594368037543));
#39352=DIRECTION('ref_axis',(2.66598427033833E-15,-0.491594368037543,0.870824309096714));
#39353=DIRECTION('',(2.66598427033951E-15,-0.491594368037543,0.870824309096714));
#39354=DIRECTION('',(1.,-5.00596043936353E-16,-3.34404360992166E-15));
#39355=DIRECTION('center_axis',(3.27370052559951E-15,0.390846788386413,
0.920455750162943));
#39356=DIRECTION('ref_axis',(8.46232198011949E-16,-0.920455750162943,0.390846788386413));
#39357=DIRECTION('',(8.46232198013806E-16,-0.920455750162943,0.390846788386413));
#39358=DIRECTION('',(1.,-5.00596043936353E-16,-3.34404360992166E-15));
#39359=DIRECTION('center_axis',(5.00596043934382E-16,1.,-5.89417440552492E-13));
#39360=DIRECTION('ref_axis',(3.34404360992196E-15,5.89417440552492E-13,
1.));
#39361=DIRECTION('',(3.34404360992225E-15,5.89417440552492E-13,1.));
#39362=DIRECTION('',(1.,-5.00596043936353E-16,-3.34404360992166E-15));
#39363=DIRECTION('center_axis',(-3.16815201654317E-15,-0.484297845738681,
-0.874903192709269));
#39364=DIRECTION('ref_axis',(-1.18154003924372E-15,0.874903192709269,-0.484297845738681));
#39365=DIRECTION('',(-1.18154003924552E-15,0.874903192709269,-0.484297845738681));
#39366=DIRECTION('center_axis',(-1.,5.00596043934459E-16,3.34404360992195E-15));
#39367=DIRECTION('ref_axis',(-5.00596043934461E-16,-1.,-6.19091607821765E-16));
#51416=CARTESIAN_POINT('',(0.,0.,0.));
#51417=CARTESIAN_POINT('Origin',(184.115917770964,-90.4720072687828,342.208039952213));
#51418=CARTESIAN_POINT('',(184.115917770964,-86.4720072687828,340.208039952213));
#51419=CARTESIAN_POINT('Origin',(184.115917770964,-90.4720072687828,340.208039952213));
#51420=CARTESIAN_POINT('',(184.115917770964,-86.4720072687828,338.208039952213));
#51421=CARTESIAN_POINT('',(184.115917770964,-86.4720072687828,342.208039952213));
#51422=CARTESIAN_POINT('Origin',(184.115917770964,-90.4720072687828,338.208039952213));
#51423=CARTESIAN_POINT('Origin',(454.115917770966,-90.4720072687829,342.208039952212));
#51424=CARTESIAN_POINT('',(454.115917770966,-86.4720072687829,340.208039952212));
#51425=CARTESIAN_POINT('Origin',(454.115917770966,-90.4720072687829,340.208039952212));
#51426=CARTESIAN_POINT('',(454.115917770966,-86.4720072687829,338.208039952212));
#51427=CARTESIAN_POINT('',(454.115917770966,-86.4720072687829,342.208039952212));
#51428=CARTESIAN_POINT('Origin',(454.115917770966,-90.4720072687829,338.208039952212));
#51429=CARTESIAN_POINT('Origin',(319.115917770965,-270.472007268783,342.208039952213));
#51430=CARTESIAN_POINT('',(319.115917770965,-266.472007268783,340.208039952213));
#51431=CARTESIAN_POINT('Origin',(319.115917770965,-270.472007268783,340.208039952213));
#51432=CARTESIAN_POINT('',(319.115917770965,-266.472007268783,338.208039952213));
#51433=CARTESIAN_POINT('',(319.115917770965,-266.472007268783,342.208039952213));
#51434=CARTESIAN_POINT('Origin',(319.115917770965,-270.472007268783,338.208039952213));
#51435=CARTESIAN_POINT('Origin',(184.115917770964,-270.472007268783,342.208039952213));
#51436=CARTESIAN_POINT('',(184.115917770964,-266.472007268783,340.208039952213));
#51437=CARTESIAN_POINT('Origin',(184.115917770964,-270.472007268783,340.208039952213));
#51438=CARTESIAN_POINT('',(184.115917770964,-266.472007268783,338.208039952213));
#51439=CARTESIAN_POINT('',(184.115917770964,-266.472007268783,342.208039952213));
#51440=CARTESIAN_POINT('Origin',(184.115917770964,-270.472007268783,338.208039952213));
#51441=CARTESIAN_POINT('Origin',(454.115917770966,-270.472007268783,342.208039952212));
#51442=CARTESIAN_POINT('',(454.115917770966,-266.472007268783,340.208039952212));
#51443=CARTESIAN_POINT('Origin',(454.115917770966,-270.472007268783,340.208039952212));
#51444=CARTESIAN_POINT('',(454.115917770966,-266.472007268783,338.208039952212));
#51445=CARTESIAN_POINT('',(454.115917770966,-266.472007268783,342.208039952212));
#51446=CARTESIAN_POINT('Origin',(454.115917770966,-270.472007268783,338.208039952212));
#51447=CARTESIAN_POINT('Origin',(319.115917770965,-90.4720072687829,342.208039952213));
#51448=CARTESIAN_POINT('',(319.115917770965,-86.4720072687829,340.208039952213));
#51449=CARTESIAN_POINT('Origin',(319.115917770965,-90.4720072687829,340.208039952213));
#51450=CARTESIAN_POINT('',(319.115917770965,-86.4720072687829,338.208039952213));
#51451=CARTESIAN_POINT('',(319.115917770965,-86.4720072687829,342.208039952213));
#51452=CARTESIAN_POINT('Origin',(319.115917770965,-90.4720072687829,338.208039952213));
#51453=CARTESIAN_POINT('Origin',(319.115917770966,-180.472007268783,338.208039952213));
#51454=CARTESIAN_POINT('',(174.115917770964,-280.472007268783,338.208039952213));
#51455=CARTESIAN_POINT('',(174.115917770964,-80.4720072687829,338.208039952213));
#51456=CARTESIAN_POINT('',(174.115917770964,-280.472007268783,338.208039952213));
#51457=CARTESIAN_POINT('',(464.115917770967,-80.472007268783,338.208039952212));
#51458=CARTESIAN_POINT('',(174.115917770964,-80.4720072687829,338.208039952213));
#51459=CARTESIAN_POINT('',(464.115917770967,-280.472007268783,338.208039952212));
#51460=CARTESIAN_POINT('',(464.115917770967,-80.472007268783,338.208039952212));
#51461=CARTESIAN_POINT('',(464.115917770967,-280.472007268783,338.208039952212));
#51462=CARTESIAN_POINT('',(444.115917770971,-99.3429750107207,338.208039952212));
#51463=CARTESIAN_POINT('',(444.115917770971,-260.472007268783,338.208039952212));
#51464=CARTESIAN_POINT('',(444.115917770971,-54.7220072688642,338.208039952212));
#51465=CARTESIAN_POINT('',(194.115917770964,-99.3429750107207,338.208039952213));
#51466=CARTESIAN_POINT('',(256.615917770965,-99.3429750107207,338.208039952213));
#51467=CARTESIAN_POINT('',(194.115917770964,-260.472007268783,338.208039952213));
#51468=CARTESIAN_POINT('',(194.115917770964,-55.8481659321689,338.208039952213));
#51469=CARTESIAN_POINT('',(256.615917770965,-260.472007268784,338.208039952213));
#51470=CARTESIAN_POINT('Origin',(464.115917770967,-280.472007268783,340.208039952212));
#51471=CARTESIAN_POINT('',(464.115917770967,-280.472007268783,340.208039952212));
#51472=CARTESIAN_POINT('',(174.115917770964,-280.472007268783,340.208039952213));
#51473=CARTESIAN_POINT('',(464.115917770967,-280.472007268783,340.208039952212));
#51474=CARTESIAN_POINT('',(174.115917770964,-280.472007268783,340.208039952213));
#51475=CARTESIAN_POINT('',(464.115917770967,-280.472007268783,340.208039952212));
#51476=CARTESIAN_POINT('Origin',(464.115917770967,-80.472007268783,340.208039952212));
#51477=CARTESIAN_POINT('',(464.115917770967,-80.472007268783,340.208039952212));
#51478=CARTESIAN_POINT('',(464.115917770967,-80.472007268783,340.208039952212));
#51479=CARTESIAN_POINT('',(464.115917770967,-80.472007268783,340.208039952212));
#51480=CARTESIAN_POINT('Origin',(174.115917770964,-80.4720072687829,340.208039952213));
#51481=CARTESIAN_POINT('',(174.115917770964,-80.4720072687829,340.208039952213));
#51482=CARTESIAN_POINT('',(174.115917770964,-80.4720072687829,340.208039952213));
#51483=CARTESIAN_POINT('',(174.115917770964,-80.4720072687829,340.208039952213));
#51484=CARTESIAN_POINT('Origin',(174.115917770964,-280.472007268783,340.208039952213));
#51485=CARTESIAN_POINT('',(174.115917770964,-280.472007268783,340.208039952213));
#51486=CARTESIAN_POINT('Origin',(194.115917770964,-260.472007268783,340.208039952213));
#51487=CARTESIAN_POINT('',(194.115917770963,-260.472007268898,154.208039952213));
#51488=CARTESIAN_POINT('',(194.115917770964,-260.472007268783,340.208039952213));
#51489=CARTESIAN_POINT('',(444.11591777097,-260.472007268898,154.208039952212));
#51490=CARTESIAN_POINT('',(194.115917770963,-260.472007268898,154.208039952213));
#51491=CARTESIAN_POINT('',(444.11591777097,-260.472007268869,201.958039952217));
#51492=CARTESIAN_POINT('Origin',(194.115917770963,68.7756754044452,71.1724431193512));
#51493=CARTESIAN_POINT('',(194.115917770963,4.52799273110809,154.208039952057));
#51494=CARTESIAN_POINT('',(194.115917770963,4.52799273110809,154.208039952057));
#51495=CARTESIAN_POINT('',(194.115917770963,402.527992731008,-14.7919600481777));
#51496=CARTESIAN_POINT('',(194.115917770963,402.527992731008,-14.7919600481777));
#51497=CARTESIAN_POINT('',(194.115917770962,402.527992730891,-212.791960048178));
#51498=CARTESIAN_POINT('',(194.115917770962,402.527992730891,-212.791960048178));
#51499=CARTESIAN_POINT('',(194.115917770963,-260.472007268898,154.208039952213));
#51500=CARTESIAN_POINT('Origin',(195.115917770993,-101.472007268812,340.208039952213));
#51501=CARTESIAN_POINT('',(443.115917770938,-101.472007268812,339.208039952212));
#51502=CARTESIAN_POINT('',(195.115917770993,-101.472007268812,339.208039952213));
#51503=CARTESIAN_POINT('',(194.615917770979,-101.472007268812,339.208039952213));
#51504=CARTESIAN_POINT('',(443.115917770938,-101.472007268812,340.208039952212));
#51505=CARTESIAN_POINT('',(443.115917770938,-101.472007268812,340.208039952212));
#51506=CARTESIAN_POINT('',(195.115917770993,-101.472007268812,340.208039952213));
#51507=CARTESIAN_POINT('',(194.615917770979,-101.472007268812,340.208039952213));
#51508=CARTESIAN_POINT('',(195.115917770993,-101.472007268812,340.208039952213));
#51509=CARTESIAN_POINT('Origin',(194.115917770964,-100.472007268783,339.208039952213));
#51510=CARTESIAN_POINT('',(195.115917770964,-101.055828398547,339.208039952213));
#51511=CARTESIAN_POINT('',(195.115917770964,-15.848165932169,339.208039952213));
#51512=CARTESIAN_POINT('',(443.115917770971,-101.055828398547,339.208039952212));
#51513=CARTESIAN_POINT('',(194.115917770964,-101.055828398547,339.208039952213));
#51514=CARTESIAN_POINT('',(443.115917770971,-14.7220072688642,339.208039952212));
#51515=CARTESIAN_POINT('Origin',(194.115917770964,-259.472007268783,340.208039952212));
#51516=CARTESIAN_POINT('',(443.115917770938,-259.472007268754,340.208039952212));
#51517=CARTESIAN_POINT('',(443.11591777097,-259.472007268898,154.797479056514));
#51518=CARTESIAN_POINT('',(443.11591777097,-259.472007268869,201.958039952216));
#51519=CARTESIAN_POINT('',(195.115917770963,-259.472007268898,154.797479056515));
#51520=CARTESIAN_POINT('',(194.115917770963,-259.472007268898,154.797479056515));
#51521=CARTESIAN_POINT('',(195.115917770993,-259.472007268754,340.208039952213));
#51522=CARTESIAN_POINT('',(195.115917770964,-259.472007268866,205.690241535883));
#51523=CARTESIAN_POINT('',(318.615917770951,-259.472007268754,340.208039952213));
#51524=CARTESIAN_POINT('Origin',(194.115917770963,3.6571684220111,153.716445584019));
#51525=CARTESIAN_POINT('',(443.11591777097,3.82426889735797,153.420439027688));
#51526=CARTESIAN_POINT('',(443.11591777097,31.063708173401,105.167718024321));
#51527=CARTESIAN_POINT('',(195.115917770963,3.82426889735809,153.420439027689));
#51528=CARTESIAN_POINT('',(195.115917770963,29.1938281577981,108.480076909111));
#51529=CARTESIAN_POINT('',(194.115917770963,3.82426889735811,153.420439027689));
#51530=CARTESIAN_POINT('Origin',(194.115917770963,402.137145942621,-15.7124157983407));
#51531=CARTESIAN_POINT('',(443.11591777097,402.527992731007,-15.8783783793395));
#51532=CARTESIAN_POINT('',(443.11591777097,247.586847758508,49.9132133301955));
#51533=CARTESIAN_POINT('',(195.115917770963,402.527992731007,-15.8783783793387));
#51534=CARTESIAN_POINT('',(195.115917770963,245.290036163702,50.8884926254802));
#51535=CARTESIAN_POINT('',(194.115917770963,402.527992731007,-15.8783783793387));
#51536=CARTESIAN_POINT('Origin',(194.115917770963,-259.98770942316,155.082943144922));
#51537=CARTESIAN_POINT('',(443.115917770969,402.527992730892,-211.648976449156));
#51538=CARTESIAN_POINT('',(443.11591777097,-113.940397936033,74.2392579023132));
#51539=CARTESIAN_POINT('',(195.115917770962,402.527992730892,-211.648976449155));
#51540=CARTESIAN_POINT('',(194.115917770962,402.527992730892,-211.648976449155));
#51541=CARTESIAN_POINT('',(195.115917770963,-116.383807447106,75.5917937855191));
#51542=CARTESIAN_POINT('Origin',(195.115917770963,68.7756754044452,71.1724431193512));
#51543=CARTESIAN_POINT('',(195.115917770963,402.527992730975,-70.8097584645117));
#51544=CARTESIAN_POINT('',(195.115917770993,-179.972007268768,340.208039952213));
#51545=CARTESIAN_POINT('Origin',(443.11591777097,71.027992731055,63.7080399520163));
#51546=CARTESIAN_POINT('',(443.11591777097,402.527992730972,-74.5419600481785));
#51547=CARTESIAN_POINT('',(443.115917770938,-100.972007268798,340.208039952212));
#51548=CARTESIAN_POINT('Origin',(194.115917770964,-100.472007268783,340.208039952213));
#51549=CARTESIAN_POINT('Origin',(194.115917770963,4.52799273110809,154.208039952057));
#51550=CARTESIAN_POINT('',(444.11591777097,4.52799273110797,154.208039952056));
#51551=CARTESIAN_POINT('',(444.11591777097,31.934532482498,105.659312392358));
#51552=CARTESIAN_POINT('',(194.115917770963,4.52799273110809,154.208039952057));
#51553=CARTESIAN_POINT('Origin',(194.115917770963,402.527992731008,-14.7919600481777));
#51554=CARTESIAN_POINT('',(444.11591777097,402.527992731008,-14.7919600481785));
#51555=CARTESIAN_POINT('',(444.11591777097,247.977694546895,50.8336690803584));
#51556=CARTESIAN_POINT('',(194.115917770963,402.527992731008,-14.7919600481777));
#51557=CARTESIAN_POINT('Origin',(194.115917770962,402.527992730891,-212.791960048178));
#51558=CARTESIAN_POINT('',(444.115917770969,402.527992730891,-212.791960048178));
#51559=CARTESIAN_POINT('',(444.11591777097,402.527992730972,-74.5419600481785));
#51560=CARTESIAN_POINT('',(194.115917770962,402.527992730891,-212.791960048178));
#51561=CARTESIAN_POINT('Origin',(194.115917770963,-260.472007268898,154.208039952213));
#51562=CARTESIAN_POINT('',(444.11591777097,-114.424695781772,73.3643547096032));
#51563=CARTESIAN_POINT('Origin',(444.11591777097,71.027992731055,63.7080399520163));
#61758=UNCERTAINTY_MEASURE_WITH_UNIT(LENGTH_MEASURE(0.01),#61812,
'DISTANCE_ACCURACY_VALUE',
'Maximum model space distance between geometric entities at asserted c
onnectivities');
#61780=UNCERTAINTY_MEASURE_WITH_UNIT(LENGTH_MEASURE(0.01),#61812,
'DISTANCE_ACCURACY_VALUE',
'Maximum model space distance between geometric entities at asserted c
onnectivities');
#61789=(
GEOMETRIC_REPRESENTATION_CONTEXT(3)
GLOBAL_UNCERTAINTY_ASSIGNED_CONTEXT((#61758))
GLOBAL_UNIT_ASSIGNED_CONTEXT((#61812,#61814,#61815))
REPRESENTATION_CONTEXT('','3D')
);
#61811=(
GEOMETRIC_REPRESENTATION_CONTEXT(3)
GLOBAL_UNCERTAINTY_ASSIGNED_CONTEXT((#61780))
GLOBAL_UNIT_ASSIGNED_CONTEXT((#61812,#61814,#61815))
REPRESENTATION_CONTEXT('','3D')
);
#61812=(
LENGTH_UNIT()
NAMED_UNIT(*)
SI_UNIT(.MILLI.,.METRE.)
);
#61814=(
NAMED_UNIT(*)
PLANE_ANGLE_UNIT()
SI_UNIT($,.RADIAN.)
);
#61815=(
NAMED_UNIT(*)
SI_UNIT($,.STERADIAN.)
SOLID_ANGLE_UNIT()
);
#61824=SHAPE_DEFINITION_REPRESENTATION(#61854,#61976);
#61854=PRODUCT_DEFINITION_SHAPE('',$,#62007);
#61976=SHAPE_REPRESENTATION('',(#34528),#61789);
#61998=PRODUCT_DEFINITION_CONTEXT('part definition',#62090,'design');
#62007=PRODUCT_DEFINITION('Discharge Chute Funnel',
'Discharge Chute Funnel',#62037,#61998);
#62037=PRODUCT_DEFINITION_FORMATION('',$,#62100);
#62090=APPLICATION_CONTEXT('Managed model based 3d engineering');
#62091=PRODUCT_CONTEXT('part definition',#62090,'mechanical');
#62100=PRODUCT('Discharge Chute Funnel','Discharge Chute Funnel',$,(#62091));
#62143=COLOUR_RGB('Sky Blue',0.24,0.69,0.87);
#62144=FILL_AREA_STYLE_COLOUR('',#62143);
#62145=FILL_AREA_STYLE('',(#62144));
#62146=SURFACE_STYLE_FILL_AREA(#62145);
#62147=SURFACE_SIDE_STYLE('',(#62146));
#62148=SURFACE_STYLE_USAGE(.BOTH.,#62147);
#62149=PRESENTATION_STYLE_ASSIGNMENT((#62148));
ENDSEC;
END-ISO-10303-21;
